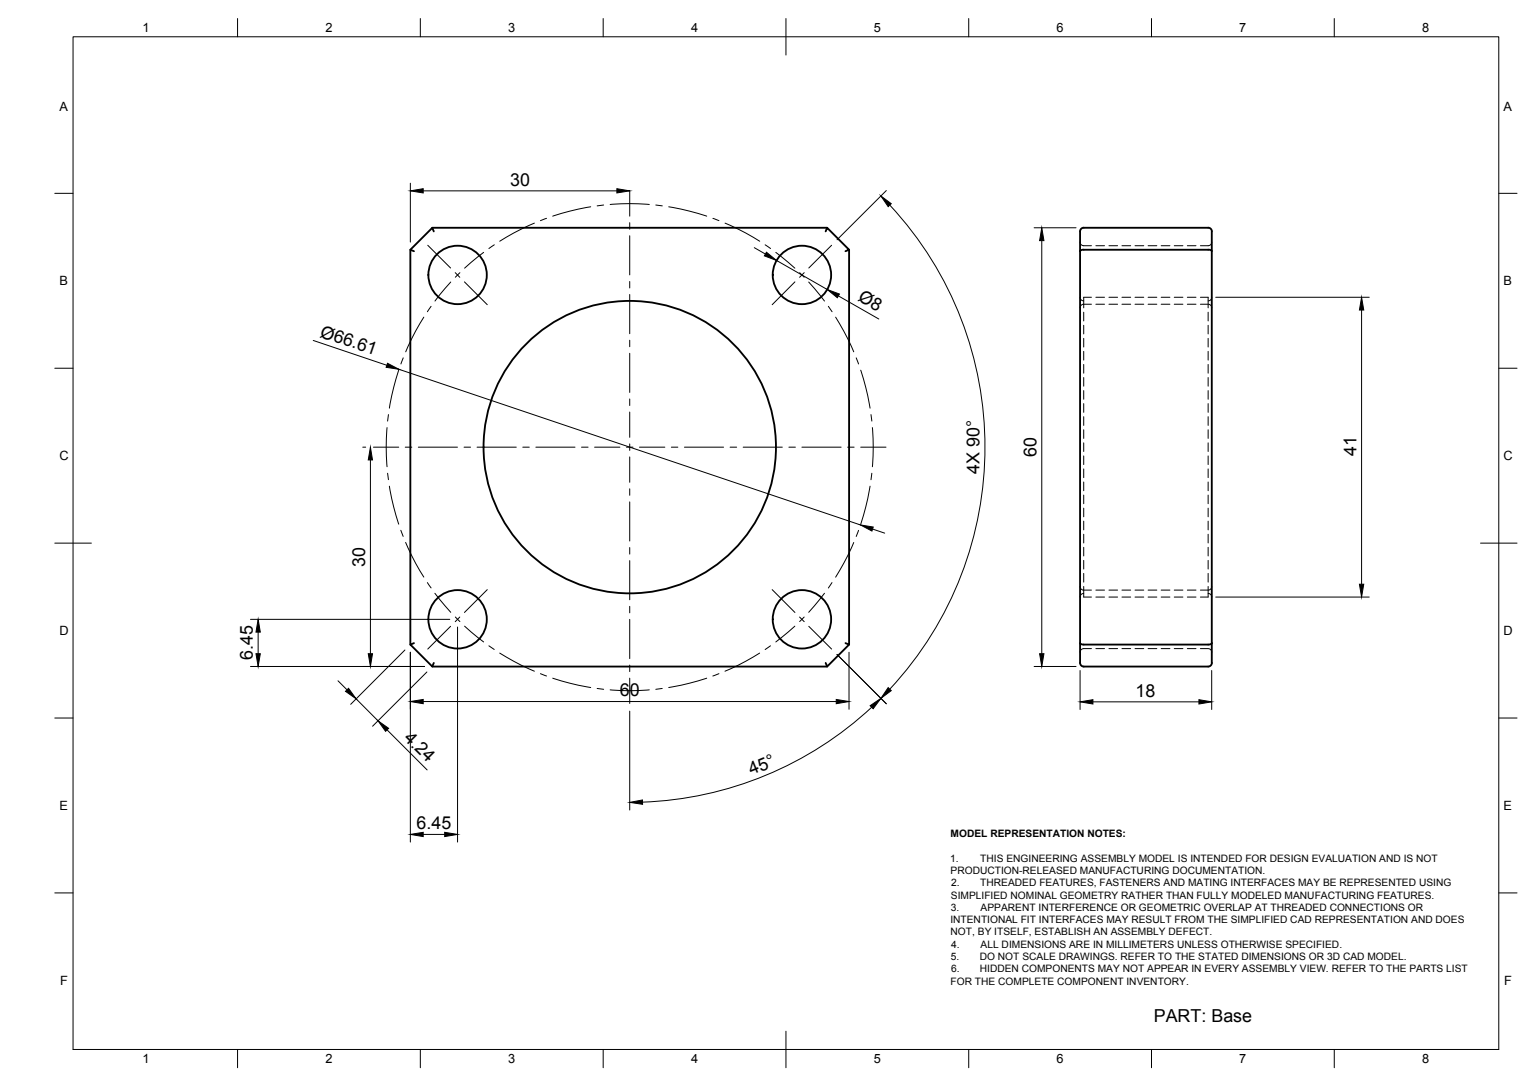
ISO-10303-21;
HEADER;
/* Generated by software containing ST-Developer
 * from STEP Tools, Inc. (www.steptools.com) 
 */

FILE_DESCRIPTION(
/* description */ (''),
/* implementation_level */ '2;1');

FILE_NAME(
/* name */ 'Base.step',
/* time_stamp */ '2026-10-05T14:32:37-07:00',
/* author */ (''),
/* organization */ (''),
/* preprocessor_version */ 'ST-DEVELOPER v20.2',
/* originating_system */ 'Autodesk Translation Framework v15.15.0.0',
/* authorisation */ '');

FILE_SCHEMA (('AUTOMOTIVE_DESIGN { 1 0 10303 214 3 1 1 }'));
ENDSEC;

DATA;
#10=MECHANICAL_DESIGN_GEOMETRIC_PRESENTATION_REPRESENTATION('',(#495),#74103);
#487=SHAPE_REPRESENTATION_RELATIONSHIP('SRR','None',#74129,#491);
#491=ADVANCED_BREP_SHAPE_REPRESENTATION('',(#499),#74100);
#495=STYLED_ITEM('',(#74157),#499);
#499=MANIFOLD_SOLID_BREP('Body1',#4574);
#512=TOROIDAL_SURFACE('',#4736,4.5,0.5);
#513=TOROIDAL_SURFACE('',#4747,4.5,0.5);
#514=TOROIDAL_SURFACE('',#4753,4.5,0.5);
#515=TOROIDAL_SURFACE('',#4759,20.5,0.5);
#516=TOROIDAL_SURFACE('',#4761,4.5,0.5);
#517=TOROIDAL_SURFACE('',#4791,4.5,0.5);
#518=TOROIDAL_SURFACE('',#4799,4.5,0.5);
#519=TOROIDAL_SURFACE('',#4801,20.5,0.5);
#520=TOROIDAL_SURFACE('',#4803,4.5,0.5);
#521=TOROIDAL_SURFACE('',#4821,4.5,0.5);
#542=ELLIPSE('',#4768,0.541196100146197,0.5);
#543=ELLIPSE('',#4769,0.541196100146199,0.5);
#544=ELLIPSE('',#4771,0.541196100146199,0.5);
#545=ELLIPSE('',#4773,0.541196100146197,0.5);
#546=ELLIPSE('',#4775,0.541196100146197,0.5);
#547=ELLIPSE('',#4776,0.541196100146197,0.5);
#548=ELLIPSE('',#4778,0.541196100146199,0.5);
#549=ELLIPSE('',#4781,0.541196100146197,0.5);
#550=ELLIPSE('',#4806,0.541196100146197,0.5);
#551=ELLIPSE('',#4807,0.541196100146198,0.5);
#552=ELLIPSE('',#4809,0.541196100146198,0.5);
#553=ELLIPSE('',#4811,0.541196100146197,0.5);
#554=ELLIPSE('',#4813,0.541196100146197,0.5);
#555=ELLIPSE('',#4814,0.541196100146197,0.5);
#556=ELLIPSE('',#4816,0.541196100146198,0.5);
#557=ELLIPSE('',#4819,0.541196100146197,0.5);
#570=FACE_BOUND('',#856,.T.);
#571=FACE_BOUND('',#858,.T.);
#572=FACE_BOUND('',#861,.T.);
#573=FACE_BOUND('',#862,.T.);
#574=FACE_BOUND('',#863,.T.);
#575=FACE_BOUND('',#864,.T.);
#576=FACE_BOUND('',#865,.T.);
#577=FACE_BOUND('',#892,.T.);
#578=FACE_BOUND('',#893,.T.);
#579=FACE_BOUND('',#894,.T.);
#580=FACE_BOUND('',#895,.T.);
#581=FACE_BOUND('',#896,.T.);
#596=PLANE('',#4730);
#597=PLANE('',#4733);
#598=PLANE('',#4740);
#599=PLANE('',#4783);
#600=PLANE('',#4784);
#601=PLANE('',#4785);
#602=PLANE('',#4786);
#603=PLANE('',#4787);
#604=PLANE('',#4788);
#605=PLANE('',#4789);
#606=PLANE('',#4790);
#607=PLANE('',#4794);
#657=FACE_OUTER_BOUND('',#855,.T.);
#658=FACE_OUTER_BOUND('',#857,.T.);
#659=FACE_OUTER_BOUND('',#859,.T.);
#660=FACE_OUTER_BOUND('',#860,.T.);
#661=FACE_OUTER_BOUND('',#866,.T.);
#662=FACE_OUTER_BOUND('',#867,.T.);
#663=FACE_OUTER_BOUND('',#868,.T.);
#664=FACE_OUTER_BOUND('',#869,.T.);
#665=FACE_OUTER_BOUND('',#870,.T.);
#666=FACE_OUTER_BOUND('',#871,.T.);
#667=FACE_OUTER_BOUND('',#872,.T.);
#668=FACE_OUTER_BOUND('',#873,.T.);
#669=FACE_OUTER_BOUND('',#874,.T.);
#670=FACE_OUTER_BOUND('',#875,.T.);
#671=FACE_OUTER_BOUND('',#876,.T.);
#672=FACE_OUTER_BOUND('',#877,.T.);
#673=FACE_OUTER_BOUND('',#878,.T.);
#674=FACE_OUTER_BOUND('',#879,.T.);
#675=FACE_OUTER_BOUND('',#880,.T.);
#676=FACE_OUTER_BOUND('',#881,.T.);
#677=FACE_OUTER_BOUND('',#882,.T.);
#678=FACE_OUTER_BOUND('',#883,.T.);
#679=FACE_OUTER_BOUND('',#884,.T.);
#680=FACE_OUTER_BOUND('',#885,.T.);
#681=FACE_OUTER_BOUND('',#886,.T.);
#682=FACE_OUTER_BOUND('',#887,.T.);
#683=FACE_OUTER_BOUND('',#888,.T.);
#684=FACE_OUTER_BOUND('',#889,.T.);
#685=FACE_OUTER_BOUND('',#890,.T.);
#686=FACE_OUTER_BOUND('',#891,.T.);
#687=FACE_OUTER_BOUND('',#897,.T.);
#688=FACE_OUTER_BOUND('',#898,.T.);
#689=FACE_OUTER_BOUND('',#899,.T.);
#690=FACE_OUTER_BOUND('',#900,.T.);
#691=FACE_OUTER_BOUND('',#901,.T.);
#692=FACE_OUTER_BOUND('',#902,.T.);
#693=FACE_OUTER_BOUND('',#903,.T.);
#694=FACE_OUTER_BOUND('',#904,.T.);
#695=FACE_OUTER_BOUND('',#905,.T.);
#696=FACE_OUTER_BOUND('',#906,.T.);
#697=FACE_OUTER_BOUND('',#907,.T.);
#698=FACE_OUTER_BOUND('',#908,.T.);
#699=FACE_OUTER_BOUND('',#909,.T.);
#855=EDGE_LOOP('',(#2985));
#856=EDGE_LOOP('',(#2986));
#857=EDGE_LOOP('',(#2987));
#858=EDGE_LOOP('',(#2988));
#859=EDGE_LOOP('',(#2989,#2990,#2991,#2992));
#860=EDGE_LOOP('',(#2993,#2994,#2995,#2996,#2997,#2998,#2999,#3000));
#861=EDGE_LOOP('',(#3001));
#862=EDGE_LOOP('',(#3002));
#863=EDGE_LOOP('',(#3003));
#864=EDGE_LOOP('',(#3004));
#865=EDGE_LOOP('',(#3005));
#866=EDGE_LOOP('',(#3006,#3007,#3008,#3009));
#867=EDGE_LOOP('',(#3010,#3011,#3012,#3013));
#868=EDGE_LOOP('',(#3014,#3015,#3016,#3017,#3018));
#869=EDGE_LOOP('',(#3019,#3020,#3021,#3022));
#870=EDGE_LOOP('',(#3023,#3024,#3025,#3026,#3027));
#871=EDGE_LOOP('',(#3028,#3029,#3030,#3031));
#872=EDGE_LOOP('',(#3032,#3033,#3034,#3035));
#873=EDGE_LOOP('',(#3036,#3037,#3038,#3039,#3040));
#874=EDGE_LOOP('',(#3041,#3042,#3043,#3044));
#875=EDGE_LOOP('',(#3045,#3046,#3047,#3048));
#876=EDGE_LOOP('',(#3049,#3050,#3051,#3052));
#877=EDGE_LOOP('',(#3053,#3054,#3055,#3056));
#878=EDGE_LOOP('',(#3057,#3058,#3059,#3060));
#879=EDGE_LOOP('',(#3061,#3062,#3063,#3064));
#880=EDGE_LOOP('',(#3065,#3066,#3067,#3068));
#881=EDGE_LOOP('',(#3069,#3070,#3071,#3072));
#882=EDGE_LOOP('',(#3073,#3074,#3075,#3076));
#883=EDGE_LOOP('',(#3077,#3078,#3079,#3080));
#884=EDGE_LOOP('',(#3081,#3082,#3083,#3084));
#885=EDGE_LOOP('',(#3085,#3086,#3087,#3088));
#886=EDGE_LOOP('',(#3089,#3090,#3091,#3092));
#887=EDGE_LOOP('',(#3093,#3094,#3095,#3096));
#888=EDGE_LOOP('',(#3097,#3098,#3099,#3100));
#889=EDGE_LOOP('',(#3101,#3102,#3103,#3104));
#890=EDGE_LOOP('',(#3105,#3106,#3107,#3108,#3109));
#891=EDGE_LOOP('',(#3110,#3111,#3112,#3113,#3114,#3115,#3116,#3117));
#892=EDGE_LOOP('',(#3118));
#893=EDGE_LOOP('',(#3119));
#894=EDGE_LOOP('',(#3120));
#895=EDGE_LOOP('',(#3121));
#896=EDGE_LOOP('',(#3122));
#897=EDGE_LOOP('',(#3123,#3124,#3125,#3126,#3127));
#898=EDGE_LOOP('',(#3128,#3129,#3130,#3131));
#899=EDGE_LOOP('',(#3132,#3133,#3134,#3135,#3136));
#900=EDGE_LOOP('',(#3137,#3138,#3139,#3140));
#901=EDGE_LOOP('',(#3141,#3142,#3143,#3144));
#902=EDGE_LOOP('',(#3145,#3146,#3147,#3148));
#903=EDGE_LOOP('',(#3149,#3150,#3151,#3152));
#904=EDGE_LOOP('',(#3153,#3154,#3155,#3156));
#905=EDGE_LOOP('',(#3157,#3158,#3159,#3160));
#906=EDGE_LOOP('',(#3161,#3162,#3163,#3164));
#907=EDGE_LOOP('',(#3165,#3166,#3167,#3168));
#908=EDGE_LOOP('',(#3169,#3170,#3171,#3172));
#909=EDGE_LOOP('',(#3173,#3174,#3175,#3176));
#1057=LINE('',#6015,#1235);
#1058=LINE('',#6017,#1236);
#1059=LINE('',#6019,#1237);
#1060=LINE('',#6021,#1238);
#1061=LINE('',#6023,#1239);
#1062=LINE('',#6025,#1240);
#1063=LINE('',#6027,#1241);
#1064=LINE('',#6028,#1242);
#1065=LINE('',#6039,#1243);
#1066=LINE('',#6047,#1244);
#1067=LINE('',#6057,#1245);
#1068=LINE('',#6069,#1246);
#1069=LINE('',#6077,#1247);
#1070=LINE('',#6082,#1248);
#1071=LINE('',#6086,#1249);
#1072=LINE('',#6091,#1250);
#1073=LINE('',#6095,#1251);
#1074=LINE('',#6098,#1252);
#1075=LINE('',#6101,#1253);
#1076=LINE('',#6104,#1254);
#1077=LINE('',#6107,#1255);
#1078=LINE('',#6109,#1256);
#1079=LINE('',#6110,#1257);
#1080=LINE('',#6113,#1258);
#1081=LINE('',#6114,#1259);
#1082=LINE('',#6117,#1260);
#1083=LINE('',#6118,#1261);
#1084=LINE('',#6121,#1262);
#1085=LINE('',#6122,#1263);
#1086=LINE('',#6125,#1264);
#1087=LINE('',#6127,#1265);
#1088=LINE('',#6128,#1266);
#1089=LINE('',#6130,#1267);
#1090=LINE('',#6133,#1268);
#1091=LINE('',#6134,#1269);
#1092=LINE('',#6136,#1270);
#1093=LINE('',#6144,#1271);
#1094=LINE('',#6146,#1272);
#1095=LINE('',#6148,#1273);
#1096=LINE('',#6150,#1274);
#1097=LINE('',#6152,#1275);
#1098=LINE('',#6154,#1276);
#1099=LINE('',#6156,#1277);
#1100=LINE('',#6157,#1278);
#1101=LINE('',#6191,#1279);
#1235=VECTOR('',#5232,10.);
#1236=VECTOR('',#5233,10.);
#1237=VECTOR('',#5234,10.);
#1238=VECTOR('',#5235,10.);
#1239=VECTOR('',#5236,10.);
#1240=VECTOR('',#5237,10.);
#1241=VECTOR('',#5238,10.);
#1242=VECTOR('',#5239,10.);
#1243=VECTOR('',#5250,4.);
#1244=VECTOR('',#5261,4.);
#1245=VECTOR('',#5274,4.);
#1246=VECTOR('',#5291,4.);
#1247=VECTOR('',#5300,9.99999999999999);
#1248=VECTOR('',#5307,10.);
#1249=VECTOR('',#5312,9.99999999999999);
#1250=VECTOR('',#5317,9.99999999999999);
#1251=VECTOR('',#5322,10.);
#1252=VECTOR('',#5327,10.);
#1253=VECTOR('',#5330,9.99999999999999);
#1254=VECTOR('',#5335,10.);
#1255=VECTOR('',#5338,10.);
#1256=VECTOR('',#5339,10.);
#1257=VECTOR('',#5340,10.);
#1258=VECTOR('',#5343,10.);
#1259=VECTOR('',#5344,9.99999999999999);
#1260=VECTOR('',#5347,10.);
#1261=VECTOR('',#5348,10.);
#1262=VECTOR('',#5351,10.);
#1263=VECTOR('',#5352,9.99999999999999);
#1264=VECTOR('',#5355,10.);
#1265=VECTOR('',#5356,9.99999999999999);
#1266=VECTOR('',#5357,10.);
#1267=VECTOR('',#5360,10.);
#1268=VECTOR('',#5363,10.);
#1269=VECTOR('',#5364,10.);
#1270=VECTOR('',#5367,9.99999999999999);
#1271=VECTOR('',#5376,10.);
#1272=VECTOR('',#5377,10.);
#1273=VECTOR('',#5378,10.);
#1274=VECTOR('',#5379,10.);
#1275=VECTOR('',#5380,10.);
#1276=VECTOR('',#5381,10.);
#1277=VECTOR('',#5382,10.);
#1278=VECTOR('',#5383,10.);
#1279=VECTOR('',#5442,20.5);
#1410=CIRCLE('',#4731,20.5);
#1411=CIRCLE('',#4732,20.);
#1412=CIRCLE('',#4734,20.5);
#1413=CIRCLE('',#4735,20.);
#1414=CIRCLE('',#4737,4.5);
#1415=CIRCLE('',#4738,0.5);
#1416=CIRCLE('',#4739,4.);
#1417=CIRCLE('',#4741,4.5);
#1418=CIRCLE('',#4742,20.5);
#1419=CIRCLE('',#4743,4.5);
#1420=CIRCLE('',#4744,4.5);
#1421=CIRCLE('',#4746,4.);
#1422=CIRCLE('',#4748,0.5);
#1423=CIRCLE('',#4749,4.);
#1424=CIRCLE('',#4751,4.);
#1425=CIRCLE('',#4752,4.);
#1426=CIRCLE('',#4754,0.5);
#1427=CIRCLE('',#4755,4.);
#1428=CIRCLE('',#4757,4.);
#1429=CIRCLE('',#4758,4.);
#1430=CIRCLE('',#4760,0.5);
#1431=CIRCLE('',#4762,0.5);
#1432=CIRCLE('',#4763,4.);
#1433=CIRCLE('',#4765,4.);
#1434=CIRCLE('',#4766,4.);
#1435=CIRCLE('',#4792,4.5);
#1436=CIRCLE('',#4793,0.5);
#1437=CIRCLE('',#4795,4.5);
#1438=CIRCLE('',#4796,4.5);
#1439=CIRCLE('',#4797,4.5);
#1440=CIRCLE('',#4798,20.5);
#1441=CIRCLE('',#4800,0.5);
#1442=CIRCLE('',#4802,0.5);
#1443=CIRCLE('',#4804,0.5);
#1444=CIRCLE('',#4822,0.5);
#1527=VERTEX_POINT('',#5997);
#1528=VERTEX_POINT('',#5999);
#1529=VERTEX_POINT('',#6002);
#1530=VERTEX_POINT('',#6004);
#1531=VERTEX_POINT('',#6007);
#1532=VERTEX_POINT('',#6009);
#1533=VERTEX_POINT('',#6013);
#1534=VERTEX_POINT('',#6014);
#1535=VERTEX_POINT('',#6016);
#1536=VERTEX_POINT('',#6018);
#1537=VERTEX_POINT('',#6020);
#1538=VERTEX_POINT('',#6022);
#1539=VERTEX_POINT('',#6024);
#1540=VERTEX_POINT('',#6026);
#1541=VERTEX_POINT('',#6029);
#1542=VERTEX_POINT('',#6031);
#1543=VERTEX_POINT('',#6033);
#1544=VERTEX_POINT('',#6035);
#1545=VERTEX_POINT('',#6038);
#1546=VERTEX_POINT('',#6042);
#1547=VERTEX_POINT('',#6046);
#1548=VERTEX_POINT('',#6048);
#1549=VERTEX_POINT('',#6052);
#1550=VERTEX_POINT('',#6056);
#1551=VERTEX_POINT('',#6058);
#1552=VERTEX_POINT('',#6064);
#1553=VERTEX_POINT('',#6068);
#1554=VERTEX_POINT('',#6070);
#1555=VERTEX_POINT('',#6074);
#1556=VERTEX_POINT('',#6076);
#1557=VERTEX_POINT('',#6080);
#1558=VERTEX_POINT('',#6084);
#1559=VERTEX_POINT('',#6088);
#1560=VERTEX_POINT('',#6090);
#1561=VERTEX_POINT('',#6094);
#1562=VERTEX_POINT('',#6100);
#1563=VERTEX_POINT('',#6106);
#1564=VERTEX_POINT('',#6108);
#1565=VERTEX_POINT('',#6112);
#1566=VERTEX_POINT('',#6116);
#1567=VERTEX_POINT('',#6120);
#1568=VERTEX_POINT('',#6124);
#1569=VERTEX_POINT('',#6126);
#1570=VERTEX_POINT('',#6132);
#1571=VERTEX_POINT('',#6138);
#1572=VERTEX_POINT('',#6142);
#1573=VERTEX_POINT('',#6143);
#1574=VERTEX_POINT('',#6145);
#1575=VERTEX_POINT('',#6147);
#1576=VERTEX_POINT('',#6149);
#1577=VERTEX_POINT('',#6151);
#1578=VERTEX_POINT('',#6153);
#1579=VERTEX_POINT('',#6155);
#1580=VERTEX_POINT('',#6158);
#1581=VERTEX_POINT('',#6160);
#1582=VERTEX_POINT('',#6162);
#1583=VERTEX_POINT('',#6164);
#2136=EDGE_CURVE('',#1527,#1527,#1410,.T.);
#2137=EDGE_CURVE('',#1528,#1528,#1411,.T.);
#2138=EDGE_CURVE('',#1529,#1529,#1412,.T.);
#2139=EDGE_CURVE('',#1530,#1530,#1413,.T.);
#2140=EDGE_CURVE('',#1531,#1531,#1414,.T.);
#2141=EDGE_CURVE('',#1531,#1532,#1415,.T.);
#2142=EDGE_CURVE('',#1532,#1532,#1416,.T.);
#2143=EDGE_CURVE('',#1533,#1534,#1057,.T.);
#2144=EDGE_CURVE('',#1535,#1533,#1058,.T.);
#2145=EDGE_CURVE('',#1536,#1535,#1059,.T.);
#2146=EDGE_CURVE('',#1537,#1536,#1060,.T.);
#2147=EDGE_CURVE('',#1538,#1537,#1061,.T.);
#2148=EDGE_CURVE('',#1539,#1538,#1062,.T.);
#2149=EDGE_CURVE('',#1540,#1539,#1063,.T.);
#2150=EDGE_CURVE('',#1534,#1540,#1064,.T.);
#2151=EDGE_CURVE('',#1541,#1541,#1417,.T.);
#2152=EDGE_CURVE('',#1542,#1542,#1418,.T.);
#2153=EDGE_CURVE('',#1543,#1543,#1419,.T.);
#2154=EDGE_CURVE('',#1544,#1544,#1420,.T.);
#2155=EDGE_CURVE('',#1532,#1545,#1065,.T.);
#2156=EDGE_CURVE('',#1545,#1545,#1421,.T.);
#2157=EDGE_CURVE('',#1541,#1546,#1422,.T.);
#2158=EDGE_CURVE('',#1546,#1546,#1423,.T.);
#2159=EDGE_CURVE('',#1546,#1547,#1066,.T.);
#2160=EDGE_CURVE('',#1548,#1547,#1424,.T.);
#2161=EDGE_CURVE('',#1547,#1548,#1425,.T.);
#2162=EDGE_CURVE('',#1544,#1549,#1426,.T.);
#2163=EDGE_CURVE('',#1549,#1549,#1427,.T.);
#2164=EDGE_CURVE('',#1549,#1550,#1067,.T.);
#2165=EDGE_CURVE('',#1551,#1550,#1428,.T.);
#2166=EDGE_CURVE('',#1550,#1551,#1429,.T.);
#2167=EDGE_CURVE('',#1542,#1528,#1430,.T.);
#2168=EDGE_CURVE('',#1543,#1552,#1431,.T.);
#2169=EDGE_CURVE('',#1552,#1552,#1432,.T.);
#2170=EDGE_CURVE('',#1552,#1553,#1068,.T.);
#2171=EDGE_CURVE('',#1554,#1553,#1433,.T.);
#2172=EDGE_CURVE('',#1553,#1554,#1434,.T.);
#2173=EDGE_CURVE('',#1537,#1555,#542,.T.);
#2174=EDGE_CURVE('',#1555,#1556,#1069,.T.);
#2175=EDGE_CURVE('',#1538,#1556,#543,.T.);
#2176=EDGE_CURVE('',#1536,#1557,#544,.T.);
#2177=EDGE_CURVE('',#1557,#1555,#1070,.T.);
#2178=EDGE_CURVE('',#1535,#1558,#545,.T.);
#2179=EDGE_CURVE('',#1558,#1557,#1071,.T.);
#2180=EDGE_CURVE('',#1534,#1559,#546,.T.);
#2181=EDGE_CURVE('',#1559,#1560,#1072,.T.);
#2182=EDGE_CURVE('',#1560,#1533,#547,.T.);
#2183=EDGE_CURVE('',#1561,#1559,#1073,.T.);
#2184=EDGE_CURVE('',#1540,#1561,#548,.T.);
#2185=EDGE_CURVE('',#1560,#1558,#1074,.T.);
#2186=EDGE_CURVE('',#1562,#1561,#1075,.T.);
#2187=EDGE_CURVE('',#1539,#1562,#549,.T.);
#2188=EDGE_CURVE('',#1556,#1562,#1076,.T.);
#2189=EDGE_CURVE('',#1557,#1563,#1077,.T.);
#2190=EDGE_CURVE('',#1564,#1563,#1078,.T.);
#2191=EDGE_CURVE('',#1555,#1564,#1079,.T.);
#2192=EDGE_CURVE('',#1558,#1565,#1080,.T.);
#2193=EDGE_CURVE('',#1563,#1565,#1081,.T.);
#2194=EDGE_CURVE('',#1560,#1566,#1082,.T.);
#2195=EDGE_CURVE('',#1565,#1566,#1083,.T.);
#2196=EDGE_CURVE('',#1559,#1567,#1084,.T.);
#2197=EDGE_CURVE('',#1566,#1567,#1085,.T.);
#2198=EDGE_CURVE('',#1562,#1568,#1086,.T.);
#2199=EDGE_CURVE('',#1569,#1568,#1087,.T.);
#2200=EDGE_CURVE('',#1561,#1569,#1088,.T.);
#2201=EDGE_CURVE('',#1567,#1569,#1089,.T.);
#2202=EDGE_CURVE('',#1556,#1570,#1090,.T.);
#2203=EDGE_CURVE('',#1568,#1570,#1091,.T.);
#2204=EDGE_CURVE('',#1570,#1564,#1092,.T.);
#2205=EDGE_CURVE('',#1571,#1571,#1435,.T.);
#2206=EDGE_CURVE('',#1571,#1548,#1436,.T.);
#2207=EDGE_CURVE('',#1572,#1573,#1093,.T.);
#2208=EDGE_CURVE('',#1574,#1572,#1094,.T.);
#2209=EDGE_CURVE('',#1575,#1574,#1095,.T.);
#2210=EDGE_CURVE('',#1576,#1575,#1096,.T.);
#2211=EDGE_CURVE('',#1577,#1576,#1097,.T.);
#2212=EDGE_CURVE('',#1578,#1577,#1098,.T.);
#2213=EDGE_CURVE('',#1579,#1578,#1099,.T.);
#2214=EDGE_CURVE('',#1573,#1579,#1100,.T.);
#2215=EDGE_CURVE('',#1580,#1580,#1437,.T.);
#2216=EDGE_CURVE('',#1581,#1581,#1438,.T.);
#2217=EDGE_CURVE('',#1582,#1582,#1439,.T.);
#2218=EDGE_CURVE('',#1583,#1583,#1440,.T.);
#2219=EDGE_CURVE('',#1580,#1551,#1441,.T.);
#2220=EDGE_CURVE('',#1583,#1530,#1442,.T.);
#2221=EDGE_CURVE('',#1581,#1554,#1443,.T.);
#2222=EDGE_CURVE('',#1576,#1563,#550,.T.);
#2223=EDGE_CURVE('',#1577,#1565,#551,.T.);
#2224=EDGE_CURVE('',#1575,#1564,#552,.T.);
#2225=EDGE_CURVE('',#1574,#1570,#553,.T.);
#2226=EDGE_CURVE('',#1573,#1569,#554,.T.);
#2227=EDGE_CURVE('',#1568,#1572,#555,.T.);
#2228=EDGE_CURVE('',#1579,#1567,#556,.T.);
#2229=EDGE_CURVE('',#1578,#1566,#557,.T.);
#2230=EDGE_CURVE('',#1545,#1582,#1444,.T.);
#2231=EDGE_CURVE('',#1527,#1529,#1101,.T.);
#2985=ORIENTED_EDGE('',*,*,#2136,.T.);
#2986=ORIENTED_EDGE('',*,*,#2137,.F.);
#2987=ORIENTED_EDGE('',*,*,#2138,.F.);
#2988=ORIENTED_EDGE('',*,*,#2139,.F.);
#2989=ORIENTED_EDGE('',*,*,#2140,.T.);
#2990=ORIENTED_EDGE('',*,*,#2141,.T.);
#2991=ORIENTED_EDGE('',*,*,#2142,.T.);
#2992=ORIENTED_EDGE('',*,*,#2141,.F.);
#2993=ORIENTED_EDGE('',*,*,#2143,.F.);
#2994=ORIENTED_EDGE('',*,*,#2144,.F.);
#2995=ORIENTED_EDGE('',*,*,#2145,.F.);
#2996=ORIENTED_EDGE('',*,*,#2146,.F.);
#2997=ORIENTED_EDGE('',*,*,#2147,.F.);
#2998=ORIENTED_EDGE('',*,*,#2148,.F.);
#2999=ORIENTED_EDGE('',*,*,#2149,.F.);
#3000=ORIENTED_EDGE('',*,*,#2150,.F.);
#3001=ORIENTED_EDGE('',*,*,#2151,.F.);
#3002=ORIENTED_EDGE('',*,*,#2152,.F.);
#3003=ORIENTED_EDGE('',*,*,#2153,.F.);
#3004=ORIENTED_EDGE('',*,*,#2154,.F.);
#3005=ORIENTED_EDGE('',*,*,#2140,.F.);
#3006=ORIENTED_EDGE('',*,*,#2142,.F.);
#3007=ORIENTED_EDGE('',*,*,#2155,.T.);
#3008=ORIENTED_EDGE('',*,*,#2156,.F.);
#3009=ORIENTED_EDGE('',*,*,#2155,.F.);
#3010=ORIENTED_EDGE('',*,*,#2151,.T.);
#3011=ORIENTED_EDGE('',*,*,#2157,.T.);
#3012=ORIENTED_EDGE('',*,*,#2158,.T.);
#3013=ORIENTED_EDGE('',*,*,#2157,.F.);
#3014=ORIENTED_EDGE('',*,*,#2158,.F.);
#3015=ORIENTED_EDGE('',*,*,#2159,.T.);
#3016=ORIENTED_EDGE('',*,*,#2160,.F.);
#3017=ORIENTED_EDGE('',*,*,#2161,.F.);
#3018=ORIENTED_EDGE('',*,*,#2159,.F.);
#3019=ORIENTED_EDGE('',*,*,#2154,.T.);
#3020=ORIENTED_EDGE('',*,*,#2162,.T.);
#3021=ORIENTED_EDGE('',*,*,#2163,.T.);
#3022=ORIENTED_EDGE('',*,*,#2162,.F.);
#3023=ORIENTED_EDGE('',*,*,#2163,.F.);
#3024=ORIENTED_EDGE('',*,*,#2164,.T.);
#3025=ORIENTED_EDGE('',*,*,#2165,.F.);
#3026=ORIENTED_EDGE('',*,*,#2166,.F.);
#3027=ORIENTED_EDGE('',*,*,#2164,.F.);
#3028=ORIENTED_EDGE('',*,*,#2152,.T.);
#3029=ORIENTED_EDGE('',*,*,#2167,.T.);
#3030=ORIENTED_EDGE('',*,*,#2137,.T.);
#3031=ORIENTED_EDGE('',*,*,#2167,.F.);
#3032=ORIENTED_EDGE('',*,*,#2153,.T.);
#3033=ORIENTED_EDGE('',*,*,#2168,.T.);
#3034=ORIENTED_EDGE('',*,*,#2169,.T.);
#3035=ORIENTED_EDGE('',*,*,#2168,.F.);
#3036=ORIENTED_EDGE('',*,*,#2169,.F.);
#3037=ORIENTED_EDGE('',*,*,#2170,.T.);
#3038=ORIENTED_EDGE('',*,*,#2171,.F.);
#3039=ORIENTED_EDGE('',*,*,#2172,.F.);
#3040=ORIENTED_EDGE('',*,*,#2170,.F.);
#3041=ORIENTED_EDGE('',*,*,#2147,.T.);
#3042=ORIENTED_EDGE('',*,*,#2173,.T.);
#3043=ORIENTED_EDGE('',*,*,#2174,.T.);
#3044=ORIENTED_EDGE('',*,*,#2175,.F.);
#3045=ORIENTED_EDGE('',*,*,#2146,.T.);
#3046=ORIENTED_EDGE('',*,*,#2176,.T.);
#3047=ORIENTED_EDGE('',*,*,#2177,.T.);
#3048=ORIENTED_EDGE('',*,*,#2173,.F.);
#3049=ORIENTED_EDGE('',*,*,#2145,.T.);
#3050=ORIENTED_EDGE('',*,*,#2178,.T.);
#3051=ORIENTED_EDGE('',*,*,#2179,.T.);
#3052=ORIENTED_EDGE('',*,*,#2176,.F.);
#3053=ORIENTED_EDGE('',*,*,#2143,.T.);
#3054=ORIENTED_EDGE('',*,*,#2180,.T.);
#3055=ORIENTED_EDGE('',*,*,#2181,.T.);
#3056=ORIENTED_EDGE('',*,*,#2182,.T.);
#3057=ORIENTED_EDGE('',*,*,#2183,.T.);
#3058=ORIENTED_EDGE('',*,*,#2180,.F.);
#3059=ORIENTED_EDGE('',*,*,#2150,.T.);
#3060=ORIENTED_EDGE('',*,*,#2184,.T.);
#3061=ORIENTED_EDGE('',*,*,#2144,.T.);
#3062=ORIENTED_EDGE('',*,*,#2182,.F.);
#3063=ORIENTED_EDGE('',*,*,#2185,.T.);
#3064=ORIENTED_EDGE('',*,*,#2178,.F.);
#3065=ORIENTED_EDGE('',*,*,#2186,.T.);
#3066=ORIENTED_EDGE('',*,*,#2184,.F.);
#3067=ORIENTED_EDGE('',*,*,#2149,.T.);
#3068=ORIENTED_EDGE('',*,*,#2187,.T.);
#3069=ORIENTED_EDGE('',*,*,#2188,.T.);
#3070=ORIENTED_EDGE('',*,*,#2187,.F.);
#3071=ORIENTED_EDGE('',*,*,#2148,.T.);
#3072=ORIENTED_EDGE('',*,*,#2175,.T.);
#3073=ORIENTED_EDGE('',*,*,#2177,.F.);
#3074=ORIENTED_EDGE('',*,*,#2189,.T.);
#3075=ORIENTED_EDGE('',*,*,#2190,.F.);
#3076=ORIENTED_EDGE('',*,*,#2191,.F.);
#3077=ORIENTED_EDGE('',*,*,#2179,.F.);
#3078=ORIENTED_EDGE('',*,*,#2192,.T.);
#3079=ORIENTED_EDGE('',*,*,#2193,.F.);
#3080=ORIENTED_EDGE('',*,*,#2189,.F.);
#3081=ORIENTED_EDGE('',*,*,#2185,.F.);
#3082=ORIENTED_EDGE('',*,*,#2194,.T.);
#3083=ORIENTED_EDGE('',*,*,#2195,.F.);
#3084=ORIENTED_EDGE('',*,*,#2192,.F.);
#3085=ORIENTED_EDGE('',*,*,#2181,.F.);
#3086=ORIENTED_EDGE('',*,*,#2196,.T.);
#3087=ORIENTED_EDGE('',*,*,#2197,.F.);
#3088=ORIENTED_EDGE('',*,*,#2194,.F.);
#3089=ORIENTED_EDGE('',*,*,#2186,.F.);
#3090=ORIENTED_EDGE('',*,*,#2198,.T.);
#3091=ORIENTED_EDGE('',*,*,#2199,.F.);
#3092=ORIENTED_EDGE('',*,*,#2200,.F.);
#3093=ORIENTED_EDGE('',*,*,#2183,.F.);
#3094=ORIENTED_EDGE('',*,*,#2200,.T.);
#3095=ORIENTED_EDGE('',*,*,#2201,.F.);
#3096=ORIENTED_EDGE('',*,*,#2196,.F.);
#3097=ORIENTED_EDGE('',*,*,#2188,.F.);
#3098=ORIENTED_EDGE('',*,*,#2202,.T.);
#3099=ORIENTED_EDGE('',*,*,#2203,.F.);
#3100=ORIENTED_EDGE('',*,*,#2198,.F.);
#3101=ORIENTED_EDGE('',*,*,#2174,.F.);
#3102=ORIENTED_EDGE('',*,*,#2191,.T.);
#3103=ORIENTED_EDGE('',*,*,#2204,.F.);
#3104=ORIENTED_EDGE('',*,*,#2202,.F.);
#3105=ORIENTED_EDGE('',*,*,#2205,.T.);
#3106=ORIENTED_EDGE('',*,*,#2206,.T.);
#3107=ORIENTED_EDGE('',*,*,#2160,.T.);
#3108=ORIENTED_EDGE('',*,*,#2161,.T.);
#3109=ORIENTED_EDGE('',*,*,#2206,.F.);
#3110=ORIENTED_EDGE('',*,*,#2207,.F.);
#3111=ORIENTED_EDGE('',*,*,#2208,.F.);
#3112=ORIENTED_EDGE('',*,*,#2209,.F.);
#3113=ORIENTED_EDGE('',*,*,#2210,.F.);
#3114=ORIENTED_EDGE('',*,*,#2211,.F.);
#3115=ORIENTED_EDGE('',*,*,#2212,.F.);
#3116=ORIENTED_EDGE('',*,*,#2213,.F.);
#3117=ORIENTED_EDGE('',*,*,#2214,.F.);
#3118=ORIENTED_EDGE('',*,*,#2215,.F.);
#3119=ORIENTED_EDGE('',*,*,#2216,.F.);
#3120=ORIENTED_EDGE('',*,*,#2217,.F.);
#3121=ORIENTED_EDGE('',*,*,#2218,.F.);
#3122=ORIENTED_EDGE('',*,*,#2205,.F.);
#3123=ORIENTED_EDGE('',*,*,#2215,.T.);
#3124=ORIENTED_EDGE('',*,*,#2219,.T.);
#3125=ORIENTED_EDGE('',*,*,#2165,.T.);
#3126=ORIENTED_EDGE('',*,*,#2166,.T.);
#3127=ORIENTED_EDGE('',*,*,#2219,.F.);
#3128=ORIENTED_EDGE('',*,*,#2218,.T.);
#3129=ORIENTED_EDGE('',*,*,#2220,.T.);
#3130=ORIENTED_EDGE('',*,*,#2139,.T.);
#3131=ORIENTED_EDGE('',*,*,#2220,.F.);
#3132=ORIENTED_EDGE('',*,*,#2216,.T.);
#3133=ORIENTED_EDGE('',*,*,#2221,.T.);
#3134=ORIENTED_EDGE('',*,*,#2171,.T.);
#3135=ORIENTED_EDGE('',*,*,#2172,.T.);
#3136=ORIENTED_EDGE('',*,*,#2221,.F.);
#3137=ORIENTED_EDGE('',*,*,#2211,.T.);
#3138=ORIENTED_EDGE('',*,*,#2222,.T.);
#3139=ORIENTED_EDGE('',*,*,#2193,.T.);
#3140=ORIENTED_EDGE('',*,*,#2223,.F.);
#3141=ORIENTED_EDGE('',*,*,#2210,.T.);
#3142=ORIENTED_EDGE('',*,*,#2224,.T.);
#3143=ORIENTED_EDGE('',*,*,#2190,.T.);
#3144=ORIENTED_EDGE('',*,*,#2222,.F.);
#3145=ORIENTED_EDGE('',*,*,#2209,.T.);
#3146=ORIENTED_EDGE('',*,*,#2225,.T.);
#3147=ORIENTED_EDGE('',*,*,#2204,.T.);
#3148=ORIENTED_EDGE('',*,*,#2224,.F.);
#3149=ORIENTED_EDGE('',*,*,#2207,.T.);
#3150=ORIENTED_EDGE('',*,*,#2226,.T.);
#3151=ORIENTED_EDGE('',*,*,#2199,.T.);
#3152=ORIENTED_EDGE('',*,*,#2227,.T.);
#3153=ORIENTED_EDGE('',*,*,#2201,.T.);
#3154=ORIENTED_EDGE('',*,*,#2226,.F.);
#3155=ORIENTED_EDGE('',*,*,#2214,.T.);
#3156=ORIENTED_EDGE('',*,*,#2228,.T.);
#3157=ORIENTED_EDGE('',*,*,#2208,.T.);
#3158=ORIENTED_EDGE('',*,*,#2227,.F.);
#3159=ORIENTED_EDGE('',*,*,#2203,.T.);
#3160=ORIENTED_EDGE('',*,*,#2225,.F.);
#3161=ORIENTED_EDGE('',*,*,#2197,.T.);
#3162=ORIENTED_EDGE('',*,*,#2228,.F.);
#3163=ORIENTED_EDGE('',*,*,#2213,.T.);
#3164=ORIENTED_EDGE('',*,*,#2229,.T.);
#3165=ORIENTED_EDGE('',*,*,#2195,.T.);
#3166=ORIENTED_EDGE('',*,*,#2229,.F.);
#3167=ORIENTED_EDGE('',*,*,#2212,.T.);
#3168=ORIENTED_EDGE('',*,*,#2223,.T.);
#3169=ORIENTED_EDGE('',*,*,#2156,.T.);
#3170=ORIENTED_EDGE('',*,*,#2230,.T.);
#3171=ORIENTED_EDGE('',*,*,#2217,.T.);
#3172=ORIENTED_EDGE('',*,*,#2230,.F.);
#3173=ORIENTED_EDGE('',*,*,#2136,.F.);
#3174=ORIENTED_EDGE('',*,*,#2231,.T.);
#3175=ORIENTED_EDGE('',*,*,#2138,.T.);
#3176=ORIENTED_EDGE('',*,*,#2231,.F.);
#4278=CYLINDRICAL_SURFACE('',#4745,4.);
#4279=CYLINDRICAL_SURFACE('',#4750,4.);
#4280=CYLINDRICAL_SURFACE('',#4756,4.);
#4281=CYLINDRICAL_SURFACE('',#4764,4.);
#4282=CYLINDRICAL_SURFACE('',#4767,0.5);
#4283=CYLINDRICAL_SURFACE('',#4770,0.5);
#4284=CYLINDRICAL_SURFACE('',#4772,0.5);
#4285=CYLINDRICAL_SURFACE('',#4774,0.5);
#4286=CYLINDRICAL_SURFACE('',#4777,0.5);
#4287=CYLINDRICAL_SURFACE('',#4779,0.5);
#4288=CYLINDRICAL_SURFACE('',#4780,0.5);
#4289=CYLINDRICAL_SURFACE('',#4782,0.5);
#4290=CYLINDRICAL_SURFACE('',#4805,0.5);
#4291=CYLINDRICAL_SURFACE('',#4808,0.5);
#4292=CYLINDRICAL_SURFACE('',#4810,0.5);
#4293=CYLINDRICAL_SURFACE('',#4812,0.5);
#4294=CYLINDRICAL_SURFACE('',#4815,0.5);
#4295=CYLINDRICAL_SURFACE('',#4817,0.5);
#4296=CYLINDRICAL_SURFACE('',#4818,0.5);
#4297=CYLINDRICAL_SURFACE('',#4820,0.5);
#4298=CYLINDRICAL_SURFACE('',#4823,20.5);
#4432=ADVANCED_FACE('',(#657,#570),#596,.F.);
#4433=ADVANCED_FACE('',(#658,#571),#597,.F.);
#4434=ADVANCED_FACE('',(#659),#512,.T.);
#4435=ADVANCED_FACE('',(#660,#572,#573,#574,#575,#576),#598,.F.);
#4436=ADVANCED_FACE('',(#661),#4278,.F.);
#4437=ADVANCED_FACE('',(#662),#513,.T.);
#4438=ADVANCED_FACE('',(#663),#4279,.F.);
#4439=ADVANCED_FACE('',(#664),#514,.T.);
#4440=ADVANCED_FACE('',(#665),#4280,.F.);
#4441=ADVANCED_FACE('',(#666),#515,.T.);
#4442=ADVANCED_FACE('',(#667),#516,.T.);
#4443=ADVANCED_FACE('',(#668),#4281,.F.);
#4444=ADVANCED_FACE('',(#669),#4282,.T.);
#4445=ADVANCED_FACE('',(#670),#4283,.T.);
#4446=ADVANCED_FACE('',(#671),#4284,.T.);
#4447=ADVANCED_FACE('',(#672),#4285,.T.);
#4448=ADVANCED_FACE('',(#673),#4286,.T.);
#4449=ADVANCED_FACE('',(#674),#4287,.T.);
#4450=ADVANCED_FACE('',(#675),#4288,.T.);
#4451=ADVANCED_FACE('',(#676),#4289,.T.);
#4452=ADVANCED_FACE('',(#677),#599,.T.);
#4453=ADVANCED_FACE('',(#678),#600,.T.);
#4454=ADVANCED_FACE('',(#679),#601,.T.);
#4455=ADVANCED_FACE('',(#680),#602,.T.);
#4456=ADVANCED_FACE('',(#681),#603,.T.);
#4457=ADVANCED_FACE('',(#682),#604,.T.);
#4458=ADVANCED_FACE('',(#683),#605,.T.);
#4459=ADVANCED_FACE('',(#684),#606,.T.);
#4460=ADVANCED_FACE('',(#685),#517,.T.);
#4461=ADVANCED_FACE('',(#686,#577,#578,#579,#580,#581),#607,.T.);
#4462=ADVANCED_FACE('',(#687),#518,.T.);
#4463=ADVANCED_FACE('',(#688),#519,.T.);
#4464=ADVANCED_FACE('',(#689),#520,.T.);
#4465=ADVANCED_FACE('',(#690),#4290,.T.);
#4466=ADVANCED_FACE('',(#691),#4291,.T.);
#4467=ADVANCED_FACE('',(#692),#4292,.T.);
#4468=ADVANCED_FACE('',(#693),#4293,.T.);
#4469=ADVANCED_FACE('',(#694),#4294,.T.);
#4470=ADVANCED_FACE('',(#695),#4295,.T.);
#4471=ADVANCED_FACE('',(#696),#4296,.T.);
#4472=ADVANCED_FACE('',(#697),#4297,.T.);
#4473=ADVANCED_FACE('',(#698),#521,.T.);
#4474=ADVANCED_FACE('',(#699),#4298,.F.);
#4574=CLOSED_SHELL('',(#4432,#4433,#4434,#4435,#4436,#4437,#4438,#4439,
#4440,#4441,#4442,#4443,#4444,#4445,#4446,#4447,#4448,#4449,#4450,#4451,
#4452,#4453,#4454,#4455,#4456,#4457,#4458,#4459,#4460,#4461,#4462,#4463,
#4464,#4465,#4466,#4467,#4468,#4469,#4470,#4471,#4472,#4473,#4474));
#4729=AXIS2_PLACEMENT_3D('',#5995,#5208,#5209);
#4730=AXIS2_PLACEMENT_3D('',#5996,#5210,#5211);
#4731=AXIS2_PLACEMENT_3D('',#5998,#5212,#5213);
#4732=AXIS2_PLACEMENT_3D('',#6000,#5214,#5215);
#4733=AXIS2_PLACEMENT_3D('',#6001,#5216,#5217);
#4734=AXIS2_PLACEMENT_3D('',#6003,#5218,#5219);
#4735=AXIS2_PLACEMENT_3D('',#6005,#5220,#5221);
#4736=AXIS2_PLACEMENT_3D('',#6006,#5222,#5223);
#4737=AXIS2_PLACEMENT_3D('',#6008,#5224,#5225);
#4738=AXIS2_PLACEMENT_3D('',#6010,#5226,#5227);
#4739=AXIS2_PLACEMENT_3D('',#6011,#5228,#5229);
#4740=AXIS2_PLACEMENT_3D('',#6012,#5230,#5231);
#4741=AXIS2_PLACEMENT_3D('',#6030,#5240,#5241);
#4742=AXIS2_PLACEMENT_3D('',#6032,#5242,#5243);
#4743=AXIS2_PLACEMENT_3D('',#6034,#5244,#5245);
#4744=AXIS2_PLACEMENT_3D('',#6036,#5246,#5247);
#4745=AXIS2_PLACEMENT_3D('',#6037,#5248,#5249);
#4746=AXIS2_PLACEMENT_3D('',#6040,#5251,#5252);
#4747=AXIS2_PLACEMENT_3D('',#6041,#5253,#5254);
#4748=AXIS2_PLACEMENT_3D('',#6043,#5255,#5256);
#4749=AXIS2_PLACEMENT_3D('',#6044,#5257,#5258);
#4750=AXIS2_PLACEMENT_3D('',#6045,#5259,#5260);
#4751=AXIS2_PLACEMENT_3D('',#6049,#5262,#5263);
#4752=AXIS2_PLACEMENT_3D('',#6050,#5264,#5265);
#4753=AXIS2_PLACEMENT_3D('',#6051,#5266,#5267);
#4754=AXIS2_PLACEMENT_3D('',#6053,#5268,#5269);
#4755=AXIS2_PLACEMENT_3D('',#6054,#5270,#5271);
#4756=AXIS2_PLACEMENT_3D('',#6055,#5272,#5273);
#4757=AXIS2_PLACEMENT_3D('',#6059,#5275,#5276);
#4758=AXIS2_PLACEMENT_3D('',#6060,#5277,#5278);
#4759=AXIS2_PLACEMENT_3D('',#6061,#5279,#5280);
#4760=AXIS2_PLACEMENT_3D('',#6062,#5281,#5282);
#4761=AXIS2_PLACEMENT_3D('',#6063,#5283,#5284);
#4762=AXIS2_PLACEMENT_3D('',#6065,#5285,#5286);
#4763=AXIS2_PLACEMENT_3D('',#6066,#5287,#5288);
#4764=AXIS2_PLACEMENT_3D('',#6067,#5289,#5290);
#4765=AXIS2_PLACEMENT_3D('',#6071,#5292,#5293);
#4766=AXIS2_PLACEMENT_3D('',#6072,#5294,#5295);
#4767=AXIS2_PLACEMENT_3D('',#6073,#5296,#5297);
#4768=AXIS2_PLACEMENT_3D('',#6075,#5298,#5299);
#4769=AXIS2_PLACEMENT_3D('',#6078,#5301,#5302);
#4770=AXIS2_PLACEMENT_3D('',#6079,#5303,#5304);
#4771=AXIS2_PLACEMENT_3D('',#6081,#5305,#5306);
#4772=AXIS2_PLACEMENT_3D('',#6083,#5308,#5309);
#4773=AXIS2_PLACEMENT_3D('',#6085,#5310,#5311);
#4774=AXIS2_PLACEMENT_3D('',#6087,#5313,#5314);
#4775=AXIS2_PLACEMENT_3D('',#6089,#5315,#5316);
#4776=AXIS2_PLACEMENT_3D('',#6092,#5318,#5319);
#4777=AXIS2_PLACEMENT_3D('',#6093,#5320,#5321);
#4778=AXIS2_PLACEMENT_3D('',#6096,#5323,#5324);
#4779=AXIS2_PLACEMENT_3D('',#6097,#5325,#5326);
#4780=AXIS2_PLACEMENT_3D('',#6099,#5328,#5329);
#4781=AXIS2_PLACEMENT_3D('',#6102,#5331,#5332);
#4782=AXIS2_PLACEMENT_3D('',#6103,#5333,#5334);
#4783=AXIS2_PLACEMENT_3D('',#6105,#5336,#5337);
#4784=AXIS2_PLACEMENT_3D('',#6111,#5341,#5342);
#4785=AXIS2_PLACEMENT_3D('',#6115,#5345,#5346);
#4786=AXIS2_PLACEMENT_3D('',#6119,#5349,#5350);
#4787=AXIS2_PLACEMENT_3D('',#6123,#5353,#5354);
#4788=AXIS2_PLACEMENT_3D('',#6129,#5358,#5359);
#4789=AXIS2_PLACEMENT_3D('',#6131,#5361,#5362);
#4790=AXIS2_PLACEMENT_3D('',#6135,#5365,#5366);
#4791=AXIS2_PLACEMENT_3D('',#6137,#5368,#5369);
#4792=AXIS2_PLACEMENT_3D('',#6139,#5370,#5371);
#4793=AXIS2_PLACEMENT_3D('',#6140,#5372,#5373);
#4794=AXIS2_PLACEMENT_3D('',#6141,#5374,#5375);
#4795=AXIS2_PLACEMENT_3D('',#6159,#5384,#5385);
#4796=AXIS2_PLACEMENT_3D('',#6161,#5386,#5387);
#4797=AXIS2_PLACEMENT_3D('',#6163,#5388,#5389);
#4798=AXIS2_PLACEMENT_3D('',#6165,#5390,#5391);
#4799=AXIS2_PLACEMENT_3D('',#6166,#5392,#5393);
#4800=AXIS2_PLACEMENT_3D('',#6167,#5394,#5395);
#4801=AXIS2_PLACEMENT_3D('',#6168,#5396,#5397);
#4802=AXIS2_PLACEMENT_3D('',#6169,#5398,#5399);
#4803=AXIS2_PLACEMENT_3D('',#6170,#5400,#5401);
#4804=AXIS2_PLACEMENT_3D('',#6171,#5402,#5403);
#4805=AXIS2_PLACEMENT_3D('',#6172,#5404,#5405);
#4806=AXIS2_PLACEMENT_3D('',#6173,#5406,#5407);
#4807=AXIS2_PLACEMENT_3D('',#6174,#5408,#5409);
#4808=AXIS2_PLACEMENT_3D('',#6175,#5410,#5411);
#4809=AXIS2_PLACEMENT_3D('',#6176,#5412,#5413);
#4810=AXIS2_PLACEMENT_3D('',#6177,#5414,#5415);
#4811=AXIS2_PLACEMENT_3D('',#6178,#5416,#5417);
#4812=AXIS2_PLACEMENT_3D('',#6179,#5418,#5419);
#4813=AXIS2_PLACEMENT_3D('',#6180,#5420,#5421);
#4814=AXIS2_PLACEMENT_3D('',#6181,#5422,#5423);
#4815=AXIS2_PLACEMENT_3D('',#6182,#5424,#5425);
#4816=AXIS2_PLACEMENT_3D('',#6183,#5426,#5427);
#4817=AXIS2_PLACEMENT_3D('',#6184,#5428,#5429);
#4818=AXIS2_PLACEMENT_3D('',#6185,#5430,#5431);
#4819=AXIS2_PLACEMENT_3D('',#6186,#5432,#5433);
#4820=AXIS2_PLACEMENT_3D('',#6187,#5434,#5435);
#4821=AXIS2_PLACEMENT_3D('',#6188,#5436,#5437);
#4822=AXIS2_PLACEMENT_3D('',#6189,#5438,#5439);
#4823=AXIS2_PLACEMENT_3D('',#6190,#5440,#5441);
#5208=DIRECTION('axis',(0.,0.,1.));
#5209=DIRECTION('refdir',(1.,0.,0.));
#5210=DIRECTION('center_axis',(0.,0.,-1.));
#5211=DIRECTION('ref_axis',(-1.,0.,0.));
#5212=DIRECTION('center_axis',(0.,0.,1.));
#5213=DIRECTION('ref_axis',(1.,0.,0.));
#5214=DIRECTION('center_axis',(0.,0.,1.));
#5215=DIRECTION('ref_axis',(1.,0.,0.));
#5216=DIRECTION('center_axis',(0.,0.,1.));
#5217=DIRECTION('ref_axis',(1.,0.,0.));
#5218=DIRECTION('center_axis',(0.,0.,1.));
#5219=DIRECTION('ref_axis',(1.,0.,0.));
#5220=DIRECTION('center_axis',(0.,0.,-1.));
#5221=DIRECTION('ref_axis',(1.,0.,0.));
#5222=DIRECTION('center_axis',(0.,0.,1.));
#5223=DIRECTION('ref_axis',(1.,0.,0.));
#5224=DIRECTION('center_axis',(0.,0.,-1.));
#5225=DIRECTION('ref_axis',(1.,0.,0.));
#5226=DIRECTION('center_axis',(0.,-1.,0.));
#5227=DIRECTION('ref_axis',(-1.,0.,0.));
#5228=DIRECTION('center_axis',(0.,0.,1.));
#5229=DIRECTION('ref_axis',(1.,0.,0.));
#5230=DIRECTION('center_axis',(0.,0.,1.));
#5231=DIRECTION('ref_axis',(1.,0.,0.));
#5232=DIRECTION('',(0.707106781186547,0.707106781186547,0.));
#5233=DIRECTION('',(1.,0.,0.));
#5234=DIRECTION('',(0.707106781186547,-0.707106781186547,0.));
#5235=DIRECTION('',(0.,-1.,0.));
#5236=DIRECTION('',(-0.707106781186547,-0.707106781186547,0.));
#5237=DIRECTION('',(-1.,0.,0.));
#5238=DIRECTION('',(-0.707106781186547,0.707106781186547,0.));
#5239=DIRECTION('',(0.,1.,0.));
#5240=DIRECTION('center_axis',(0.,0.,-1.));
#5241=DIRECTION('ref_axis',(1.,0.,0.));
#5242=DIRECTION('center_axis',(0.,0.,-1.));
#5243=DIRECTION('ref_axis',(1.,0.,0.));
#5244=DIRECTION('center_axis',(0.,0.,-1.));
#5245=DIRECTION('ref_axis',(1.,0.,0.));
#5246=DIRECTION('center_axis',(0.,0.,-1.));
#5247=DIRECTION('ref_axis',(1.,0.,0.));
#5248=DIRECTION('center_axis',(0.,0.,1.));
#5249=DIRECTION('ref_axis',(1.,0.,0.));
#5250=DIRECTION('',(0.,0.,1.));
#5251=DIRECTION('center_axis',(0.,0.,-1.));
#5252=DIRECTION('ref_axis',(1.,0.,0.));
#5253=DIRECTION('center_axis',(0.,0.,1.));
#5254=DIRECTION('ref_axis',(1.,0.,0.));
#5255=DIRECTION('center_axis',(0.,-1.,0.));
#5256=DIRECTION('ref_axis',(-1.,0.,0.));
#5257=DIRECTION('center_axis',(0.,0.,1.));
#5258=DIRECTION('ref_axis',(1.,0.,0.));
#5259=DIRECTION('center_axis',(0.,0.,1.));
#5260=DIRECTION('ref_axis',(1.,0.,0.));
#5261=DIRECTION('',(0.,0.,1.));
#5262=DIRECTION('center_axis',(0.,0.,-1.));
#5263=DIRECTION('ref_axis',(1.,0.,0.));
#5264=DIRECTION('center_axis',(0.,0.,-1.));
#5265=DIRECTION('ref_axis',(1.,0.,0.));
#5266=DIRECTION('center_axis',(0.,0.,1.));
#5267=DIRECTION('ref_axis',(1.,0.,0.));
#5268=DIRECTION('center_axis',(0.,-1.,0.));
#5269=DIRECTION('ref_axis',(-1.,0.,0.));
#5270=DIRECTION('center_axis',(0.,0.,1.));
#5271=DIRECTION('ref_axis',(1.,0.,0.));
#5272=DIRECTION('center_axis',(0.,0.,1.));
#5273=DIRECTION('ref_axis',(1.,0.,0.));
#5274=DIRECTION('',(0.,0.,1.));
#5275=DIRECTION('center_axis',(0.,0.,-1.));
#5276=DIRECTION('ref_axis',(1.,0.,0.));
#5277=DIRECTION('center_axis',(0.,0.,-1.));
#5278=DIRECTION('ref_axis',(1.,0.,0.));
#5279=DIRECTION('center_axis',(0.,0.,1.));
#5280=DIRECTION('ref_axis',(1.,0.,0.));
#5281=DIRECTION('center_axis',(1.22464679914735E-16,-1.,0.));
#5282=DIRECTION('ref_axis',(-1.,-1.22464679914735E-16,0.));
#5283=DIRECTION('center_axis',(0.,0.,1.));
#5284=DIRECTION('ref_axis',(1.,0.,0.));
#5285=DIRECTION('center_axis',(0.,-1.,0.));
#5286=DIRECTION('ref_axis',(-1.,0.,0.));
#5287=DIRECTION('center_axis',(0.,0.,1.));
#5288=DIRECTION('ref_axis',(1.,0.,0.));
#5289=DIRECTION('center_axis',(0.,0.,1.));
#5290=DIRECTION('ref_axis',(1.,0.,0.));
#5291=DIRECTION('',(0.,0.,1.));
#5292=DIRECTION('center_axis',(0.,0.,-1.));
#5293=DIRECTION('ref_axis',(1.,0.,0.));
#5294=DIRECTION('center_axis',(0.,0.,-1.));
#5295=DIRECTION('ref_axis',(1.,0.,0.));
#5296=DIRECTION('center_axis',(0.707106781186548,0.707106781186548,0.));
#5297=DIRECTION('ref_axis',(-0.499999999999996,0.499999999999996,-0.707106781186553));
#5298=DIRECTION('center_axis',(0.382683432365092,0.923879532511286,0.));
#5299=DIRECTION('ref_axis',(-0.923879532511286,0.382683432365092,0.));
#5300=DIRECTION('',(0.707106781186547,0.707106781186547,0.));
#5301=DIRECTION('center_axis',(0.923879532511283,0.382683432365099,3.39891166203448E-15));
#5302=DIRECTION('ref_axis',(-0.382683432365099,0.923879532511283,8.2056986317915E-15));
#5303=DIRECTION('center_axis',(0.,1.,0.));
#5304=DIRECTION('ref_axis',(-0.707106781186541,0.,-0.707106781186554));
#5305=DIRECTION('center_axis',(-0.382683432365099,0.923879532511283,3.39891166203448E-15));
#5306=DIRECTION('ref_axis',(-0.923879532511283,-0.382683432365099,8.2056986317915E-15));
#5307=DIRECTION('',(0.,1.,0.));
#5308=DIRECTION('center_axis',(-0.707106781186548,0.707106781186548,0.));
#5309=DIRECTION('ref_axis',(-0.499999999999996,-0.499999999999996,-0.707106781186553));
#5310=DIRECTION('center_axis',(-0.923879532511286,0.382683432365092,0.));
#5311=DIRECTION('ref_axis',(-0.382683432365092,-0.923879532511286,0.));
#5312=DIRECTION('',(-0.707106781186547,0.707106781186547,0.));
#5313=DIRECTION('center_axis',(-0.707106781186548,-0.707106781186548,0.));
#5314=DIRECTION('ref_axis',(0.499999999999996,-0.499999999999996,-0.707106781186553));
#5315=DIRECTION('center_axis',(-0.382683432365092,-0.923879532511286,0.));
#5316=DIRECTION('ref_axis',(0.923879532511286,-0.382683432365092,0.));
#5317=DIRECTION('',(-0.707106781186547,-0.707106781186547,0.));
#5318=DIRECTION('center_axis',(0.923879532511286,0.382683432365092,-8.20569863179153E-15));
#5319=DIRECTION('ref_axis',(-0.382683432365092,0.923879532511286,1.98103089256176E-14));
#5320=DIRECTION('center_axis',(0.,-1.,0.));
#5321=DIRECTION('ref_axis',(0.707106781186541,0.,-0.707106781186554));
#5322=DIRECTION('',(0.,-1.,0.));
#5323=DIRECTION('center_axis',(0.382683432365099,-0.923879532511283,3.39891166203448E-15));
#5324=DIRECTION('ref_axis',(0.923879532511283,0.382683432365099,8.2056986317915E-15));
#5325=DIRECTION('center_axis',(-1.,0.,0.));
#5326=DIRECTION('ref_axis',(0.,-0.707106781186541,-0.707106781186554));
#5327=DIRECTION('',(-1.,0.,0.));
#5328=DIRECTION('center_axis',(0.707106781186548,-0.707106781186548,0.));
#5329=DIRECTION('ref_axis',(0.499999999999996,0.499999999999996,-0.707106781186553));
#5330=DIRECTION('',(0.707106781186547,-0.707106781186547,0.));
#5331=DIRECTION('center_axis',(0.923879532511286,-0.382683432365092,0.));
#5332=DIRECTION('ref_axis',(0.382683432365092,0.923879532511286,0.));
#5333=DIRECTION('center_axis',(1.,0.,0.));
#5334=DIRECTION('ref_axis',(0.,0.707106781186541,-0.707106781186554));
#5335=DIRECTION('',(1.,0.,0.));
#5336=DIRECTION('center_axis',(-1.,0.,0.));
#5337=DIRECTION('ref_axis',(0.,-1.,0.));
#5338=DIRECTION('',(0.,0.,1.));
#5339=DIRECTION('',(0.,-1.,0.));
#5340=DIRECTION('',(0.,0.,1.));
#5341=DIRECTION('center_axis',(-0.707106781186548,-0.707106781186548,0.));
#5342=DIRECTION('ref_axis',(0.707106781186548,-0.707106781186548,0.));
#5343=DIRECTION('',(0.,0.,1.));
#5344=DIRECTION('',(0.707106781186547,-0.707106781186547,0.));
#5345=DIRECTION('center_axis',(0.,-1.,0.));
#5346=DIRECTION('ref_axis',(1.,0.,0.));
#5347=DIRECTION('',(0.,0.,1.));
#5348=DIRECTION('',(1.,0.,0.));
#5349=DIRECTION('center_axis',(0.707106781186548,-0.707106781186548,0.));
#5350=DIRECTION('ref_axis',(0.707106781186548,0.707106781186548,0.));
#5351=DIRECTION('',(0.,0.,1.));
#5352=DIRECTION('',(0.707106781186547,0.707106781186547,0.));
#5353=DIRECTION('center_axis',(0.707106781186548,0.707106781186548,0.));
#5354=DIRECTION('ref_axis',(-0.707106781186548,0.707106781186548,0.));
#5355=DIRECTION('',(0.,0.,1.));
#5356=DIRECTION('',(-0.707106781186547,0.707106781186547,0.));
#5357=DIRECTION('',(0.,0.,1.));
#5358=DIRECTION('center_axis',(1.,0.,0.));
#5359=DIRECTION('ref_axis',(0.,1.,0.));
#5360=DIRECTION('',(0.,1.,0.));
#5361=DIRECTION('center_axis',(0.,1.,0.));
#5362=DIRECTION('ref_axis',(-1.,0.,0.));
#5363=DIRECTION('',(0.,0.,1.));
#5364=DIRECTION('',(-1.,0.,0.));
#5365=DIRECTION('center_axis',(-0.707106781186548,0.707106781186548,0.));
#5366=DIRECTION('ref_axis',(-0.707106781186548,-0.707106781186548,0.));
#5367=DIRECTION('',(-0.707106781186547,-0.707106781186547,0.));
#5368=DIRECTION('center_axis',(0.,0.,-1.));
#5369=DIRECTION('ref_axis',(-1.,0.,0.));
#5370=DIRECTION('center_axis',(0.,0.,1.));
#5371=DIRECTION('ref_axis',(1.,0.,0.));
#5372=DIRECTION('center_axis',(0.,-1.,0.));
#5373=DIRECTION('ref_axis',(1.,0.,0.));
#5374=DIRECTION('center_axis',(0.,0.,1.));
#5375=DIRECTION('ref_axis',(1.,0.,0.));
#5376=DIRECTION('',(0.707106781186547,-0.707106781186547,0.));
#5377=DIRECTION('',(1.,0.,0.));
#5378=DIRECTION('',(0.707106781186547,0.707106781186547,0.));
#5379=DIRECTION('',(0.,1.,0.));
#5380=DIRECTION('',(-0.707106781186547,0.707106781186547,0.));
#5381=DIRECTION('',(-1.,0.,0.));
#5382=DIRECTION('',(-0.707106781186547,-0.707106781186547,0.));
#5383=DIRECTION('',(0.,-1.,0.));
#5384=DIRECTION('center_axis',(0.,0.,1.));
#5385=DIRECTION('ref_axis',(1.,0.,0.));
#5386=DIRECTION('center_axis',(0.,0.,1.));
#5387=DIRECTION('ref_axis',(1.,0.,0.));
#5388=DIRECTION('center_axis',(0.,0.,1.));
#5389=DIRECTION('ref_axis',(1.,0.,0.));
#5390=DIRECTION('center_axis',(0.,0.,1.));
#5391=DIRECTION('ref_axis',(1.,0.,0.));
#5392=DIRECTION('center_axis',(0.,0.,-1.));
#5393=DIRECTION('ref_axis',(-1.,0.,0.));
#5394=DIRECTION('center_axis',(0.,-1.,0.));
#5395=DIRECTION('ref_axis',(1.,0.,0.));
#5396=DIRECTION('center_axis',(0.,0.,-1.));
#5397=DIRECTION('ref_axis',(-1.,0.,0.));
#5398=DIRECTION('center_axis',(-1.22464679914735E-16,-1.,0.));
#5399=DIRECTION('ref_axis',(1.,-1.22464679914735E-16,0.));
#5400=DIRECTION('center_axis',(0.,0.,-1.));
#5401=DIRECTION('ref_axis',(-1.,0.,0.));
#5402=DIRECTION('center_axis',(0.,-1.,0.));
#5403=DIRECTION('ref_axis',(1.,0.,0.));
#5404=DIRECTION('center_axis',(0.707106781186548,-0.707106781186548,0.));
#5405=DIRECTION('ref_axis',(-0.5,-0.5,0.707106781186547));
#5406=DIRECTION('center_axis',(0.382683432365092,-0.923879532511286,8.20569863179167E-15));
#5407=DIRECTION('ref_axis',(-0.923879532511286,-0.382683432365092,1.98103089256179E-14));
#5408=DIRECTION('center_axis',(0.923879532511286,-0.382683432365092,0.));
#5409=DIRECTION('ref_axis',(-0.382683432365092,-0.923879532511286,0.));
#5410=DIRECTION('center_axis',(0.,-1.,0.));
#5411=DIRECTION('ref_axis',(-0.707106781186548,0.,0.707106781186548));
#5412=DIRECTION('center_axis',(-0.382683432365092,-0.923879532511286,0.));
#5413=DIRECTION('ref_axis',(-0.923879532511286,0.382683432365092,0.));
#5414=DIRECTION('center_axis',(-0.707106781186548,-0.707106781186548,0.));
#5415=DIRECTION('ref_axis',(-0.5,0.5,0.707106781186547));
#5416=DIRECTION('center_axis',(-0.923879532511286,-0.382683432365092,8.20569863179167E-15));
#5417=DIRECTION('ref_axis',(-0.382683432365092,0.923879532511286,1.98103089256179E-14));
#5418=DIRECTION('center_axis',(-0.707106781186548,0.707106781186548,0.));
#5419=DIRECTION('ref_axis',(0.5,0.5,0.707106781186547));
#5420=DIRECTION('center_axis',(-0.382683432365092,0.923879532511286,8.20569863179167E-15));
#5421=DIRECTION('ref_axis',(0.923879532511286,0.382683432365092,1.98103089256179E-14));
#5422=DIRECTION('center_axis',(0.923879532511286,-0.382683432365092,0.));
#5423=DIRECTION('ref_axis',(-0.382683432365092,-0.923879532511286,0.));
#5424=DIRECTION('center_axis',(0.,1.,0.));
#5425=DIRECTION('ref_axis',(0.707106781186548,0.,0.707106781186548));
#5426=DIRECTION('center_axis',(0.382683432365092,0.923879532511286,0.));
#5427=DIRECTION('ref_axis',(0.923879532511286,-0.382683432365092,0.));
#5428=DIRECTION('center_axis',(-1.,0.,0.));
#5429=DIRECTION('ref_axis',(0.,0.707106781186548,0.707106781186548));
#5430=DIRECTION('center_axis',(0.707106781186548,0.707106781186548,0.));
#5431=DIRECTION('ref_axis',(0.5,-0.5,0.707106781186547));
#5432=DIRECTION('center_axis',(0.923879532511286,0.382683432365092,8.20569863179167E-15));
#5433=DIRECTION('ref_axis',(0.382683432365092,-0.923879532511286,1.98103089256179E-14));
#5434=DIRECTION('center_axis',(1.,0.,0.));
#5435=DIRECTION('ref_axis',(0.,-0.707106781186548,0.707106781186548));
#5436=DIRECTION('center_axis',(0.,0.,1.));
#5437=DIRECTION('ref_axis',(1.,0.,0.));
#5438=DIRECTION('center_axis',(0.,-1.,0.));
#5439=DIRECTION('ref_axis',(-1.,0.,0.));
#5440=DIRECTION('center_axis',(0.,0.,1.));
#5441=DIRECTION('ref_axis',(1.,0.,0.));
#5442=DIRECTION('',(0.,0.,1.));
#5995=CARTESIAN_POINT('',(0.,0.,0.));
#5996=CARTESIAN_POINT('Origin',(20.5,0.,-54.5));
#5997=CARTESIAN_POINT('',(-20.5,-2.51052593825207E-15,-54.5));
#5998=CARTESIAN_POINT('Origin',(0.,0.,-54.5));
#5999=CARTESIAN_POINT('',(-20.,-2.44929359829471E-15,-54.5));
#6000=CARTESIAN_POINT('Origin',(0.,0.,-54.5));
#6001=CARTESIAN_POINT('Origin',(20.,0.,-37.5));
#6002=CARTESIAN_POINT('',(-20.5,-2.51052593825207E-15,-37.5));
#6003=CARTESIAN_POINT('Origin',(0.,0.,-37.5));
#6004=CARTESIAN_POINT('',(20.,-2.44929359829471E-15,-37.5));
#6005=CARTESIAN_POINT('Origin',(0.,0.,-37.5));
#6006=CARTESIAN_POINT('Origin',(23.5502525316942,-23.5502525316942,-54.5));
#6007=CARTESIAN_POINT('',(19.0502525316942,-23.5502525316942,-55.));
#6008=CARTESIAN_POINT('Origin',(23.5502525316942,-23.5502525316942,-55.));
#6009=CARTESIAN_POINT('',(19.5502525316942,-23.5502525316942,-54.5));
#6010=CARTESIAN_POINT('Origin',(19.0502525316942,-23.5502525316942,-54.5));
#6011=CARTESIAN_POINT('Origin',(23.5502525316942,-23.5502525316942,-54.5));
#6012=CARTESIAN_POINT('Origin',(0.,0.,-55.));
#6013=CARTESIAN_POINT('',(26.7928932188135,-29.5,-55.));
#6014=CARTESIAN_POINT('',(29.5,-26.7928932188135,-55.));
#6015=CARTESIAN_POINT('',(27.3964466094067,-28.8964466094067,-55.));
#6016=CARTESIAN_POINT('',(-26.7928932188135,-29.5,-55.));
#6017=CARTESIAN_POINT('',(-13.5,-29.5,-55.));
#6018=CARTESIAN_POINT('',(-29.5,-26.7928932188135,-55.));
#6019=CARTESIAN_POINT('',(-28.8964466094067,-27.3964466094067,-55.));
#6020=CARTESIAN_POINT('',(-29.5,26.7928932188135,-55.));
#6021=CARTESIAN_POINT('',(-29.5,13.5,-55.));
#6022=CARTESIAN_POINT('',(-26.7928932188135,29.5,-55.));
#6023=CARTESIAN_POINT('',(-27.3964466094067,28.8964466094067,-55.));
#6024=CARTESIAN_POINT('',(26.7928932188135,29.5,-55.));
#6025=CARTESIAN_POINT('',(13.5,29.5,-55.));
#6026=CARTESIAN_POINT('',(29.5,26.7928932188135,-55.));
#6027=CARTESIAN_POINT('',(28.8964466094067,27.3964466094067,-55.));
#6028=CARTESIAN_POINT('',(29.5,-13.5,-55.));
#6029=CARTESIAN_POINT('',(-28.0502525316942,23.5502525316942,-55.));
#6030=CARTESIAN_POINT('Origin',(-23.5502525316942,23.5502525316942,-55.));
#6031=CARTESIAN_POINT('',(-20.5,2.51052593825207E-15,-55.));
#6032=CARTESIAN_POINT('Origin',(0.,0.,-55.));
#6033=CARTESIAN_POINT('',(19.0502525316942,23.5502525316942,-55.));
#6034=CARTESIAN_POINT('Origin',(23.5502525316942,23.5502525316942,-55.));
#6035=CARTESIAN_POINT('',(-28.0502525316942,-23.5502525316942,-55.));
#6036=CARTESIAN_POINT('Origin',(-23.5502525316942,-23.5502525316942,-55.));
#6037=CARTESIAN_POINT('Origin',(23.5502525316942,-23.5502525316942,-50.));
#6038=CARTESIAN_POINT('',(19.5502525316942,-23.5502525316942,-37.5));
#6039=CARTESIAN_POINT('',(19.5502525316942,-23.5502525316942,-50.));
#6040=CARTESIAN_POINT('Origin',(23.5502525316942,-23.5502525316942,-37.5));
#6041=CARTESIAN_POINT('Origin',(-23.5502525316942,23.5502525316942,-54.5));
#6042=CARTESIAN_POINT('',(-27.5502525316942,23.5502525316942,-54.5));
#6043=CARTESIAN_POINT('Origin',(-28.0502525316942,23.5502525316942,-54.5));
#6044=CARTESIAN_POINT('Origin',(-23.5502525316942,23.5502525316942,-54.5));
#6045=CARTESIAN_POINT('Origin',(-23.5502525316942,23.5502525316942,-50.));
#6046=CARTESIAN_POINT('',(-27.5502525316942,23.5502525316942,-37.5));
#6047=CARTESIAN_POINT('',(-27.5502525316942,23.5502525316942,-50.));
#6048=CARTESIAN_POINT('',(-19.5502525316942,23.5502525316942,-37.5));
#6049=CARTESIAN_POINT('Origin',(-23.5502525316942,23.5502525316942,-37.5));
#6050=CARTESIAN_POINT('Origin',(-23.5502525316942,23.5502525316942,-37.5));
#6051=CARTESIAN_POINT('Origin',(-23.5502525316942,-23.5502525316942,-54.5));
#6052=CARTESIAN_POINT('',(-27.5502525316942,-23.5502525316942,-54.5));
#6053=CARTESIAN_POINT('Origin',(-28.0502525316942,-23.5502525316942,-54.5));
#6054=CARTESIAN_POINT('Origin',(-23.5502525316942,-23.5502525316942,-54.5));
#6055=CARTESIAN_POINT('Origin',(-23.5502525316942,-23.5502525316942,-50.));
#6056=CARTESIAN_POINT('',(-27.5502525316942,-23.5502525316942,-37.5));
#6057=CARTESIAN_POINT('',(-27.5502525316942,-23.5502525316942,-50.));
#6058=CARTESIAN_POINT('',(-19.5502525316942,-23.5502525316942,-37.5));
#6059=CARTESIAN_POINT('Origin',(-23.5502525316942,-23.5502525316942,-37.5));
#6060=CARTESIAN_POINT('Origin',(-23.5502525316942,-23.5502525316942,-37.5));
#6061=CARTESIAN_POINT('Origin',(0.,0.,-54.5));
#6062=CARTESIAN_POINT('Origin',(-20.5,-2.51052593825207E-15,-54.5));
#6063=CARTESIAN_POINT('Origin',(23.5502525316942,23.5502525316942,-54.5));
#6064=CARTESIAN_POINT('',(19.5502525316942,23.5502525316942,-54.5));
#6065=CARTESIAN_POINT('Origin',(19.0502525316942,23.5502525316942,-54.5));
#6066=CARTESIAN_POINT('Origin',(23.5502525316942,23.5502525316942,-54.5));
#6067=CARTESIAN_POINT('Origin',(23.5502525316942,23.5502525316942,-50.));
#6068=CARTESIAN_POINT('',(19.5502525316942,23.5502525316942,-37.5));
#6069=CARTESIAN_POINT('',(19.5502525316942,23.5502525316942,-50.));
#6070=CARTESIAN_POINT('',(27.5502525316942,23.5502525316942,-37.5));
#6071=CARTESIAN_POINT('Origin',(23.5502525316942,23.5502525316942,-37.5));
#6072=CARTESIAN_POINT('Origin',(23.5502525316942,23.5502525316942,-37.5));
#6073=CARTESIAN_POINT('Origin',(-27.3964466094067,28.8964466094067,-54.5));
#6074=CARTESIAN_POINT('',(-30.,27.,-54.5));
#6075=CARTESIAN_POINT('Origin',(-29.5,26.7928932188135,-54.5));
#6076=CARTESIAN_POINT('',(-27.,30.,-54.5));
#6077=CARTESIAN_POINT('',(-27.75,29.25,-54.5));
#6078=CARTESIAN_POINT('Origin',(-26.7928932188135,29.5,-54.5));
#6079=CARTESIAN_POINT('Origin',(-29.5,13.5,-54.5));
#6080=CARTESIAN_POINT('',(-30.,-27.,-54.5));
#6081=CARTESIAN_POINT('Origin',(-29.5,-26.7928932188135,-54.5));
#6082=CARTESIAN_POINT('',(-30.,13.5,-54.5));
#6083=CARTESIAN_POINT('Origin',(-28.8964466094067,-27.3964466094067,-54.5));
#6084=CARTESIAN_POINT('',(-27.,-30.,-54.5));
#6085=CARTESIAN_POINT('Origin',(-26.7928932188135,-29.5,-54.5));
#6086=CARTESIAN_POINT('',(-29.25,-27.75,-54.5));
#6087=CARTESIAN_POINT('Origin',(27.3964466094067,-28.8964466094067,-54.5));
#6088=CARTESIAN_POINT('',(30.,-27.,-54.5));
#6089=CARTESIAN_POINT('Origin',(29.5,-26.7928932188135,-54.5));
#6090=CARTESIAN_POINT('',(27.,-30.,-54.5));
#6091=CARTESIAN_POINT('',(27.75,-29.25,-54.5));
#6092=CARTESIAN_POINT('Origin',(26.7928932188135,-29.5,-54.5));
#6093=CARTESIAN_POINT('Origin',(29.5,-13.5,-54.5));
#6094=CARTESIAN_POINT('',(30.,27.,-54.5));
#6095=CARTESIAN_POINT('',(30.,-13.5,-54.5));
#6096=CARTESIAN_POINT('Origin',(29.5,26.7928932188135,-54.5));
#6097=CARTESIAN_POINT('Origin',(-13.5,-29.5,-54.5));
#6098=CARTESIAN_POINT('',(-13.5,-30.,-54.5));
#6099=CARTESIAN_POINT('Origin',(28.8964466094067,27.3964466094067,-54.5));
#6100=CARTESIAN_POINT('',(27.,30.,-54.5));
#6101=CARTESIAN_POINT('',(29.25,27.75,-54.5));
#6102=CARTESIAN_POINT('Origin',(26.7928932188135,29.5,-54.5));
#6103=CARTESIAN_POINT('Origin',(13.5,29.5,-54.5));
#6104=CARTESIAN_POINT('',(13.5,30.,-54.5));
#6105=CARTESIAN_POINT('Origin',(-30.,27.,-50.));
#6106=CARTESIAN_POINT('',(-30.,-27.,-37.5));
#6107=CARTESIAN_POINT('',(-30.,-27.,-50.));
#6108=CARTESIAN_POINT('',(-30.,27.,-37.5));
#6109=CARTESIAN_POINT('',(-30.,13.5,-37.5));
#6110=CARTESIAN_POINT('',(-30.,27.,-50.));
#6111=CARTESIAN_POINT('Origin',(-30.,-27.,-50.));
#6112=CARTESIAN_POINT('',(-27.,-30.,-37.5));
#6113=CARTESIAN_POINT('',(-27.,-30.,-50.));
#6114=CARTESIAN_POINT('',(-29.25,-27.75,-37.5));
#6115=CARTESIAN_POINT('Origin',(-27.,-30.,-50.));
#6116=CARTESIAN_POINT('',(27.,-30.,-37.5));
#6117=CARTESIAN_POINT('',(27.,-30.,-50.));
#6118=CARTESIAN_POINT('',(-13.5,-30.,-37.5));
#6119=CARTESIAN_POINT('Origin',(27.,-30.,-50.));
#6120=CARTESIAN_POINT('',(30.,-27.,-37.5));
#6121=CARTESIAN_POINT('',(30.,-27.,-50.));
#6122=CARTESIAN_POINT('',(27.75,-29.25,-37.5));
#6123=CARTESIAN_POINT('Origin',(30.,27.,-50.));
#6124=CARTESIAN_POINT('',(27.,30.,-37.5));
#6125=CARTESIAN_POINT('',(27.,30.,-50.));
#6126=CARTESIAN_POINT('',(30.,27.,-37.5));
#6127=CARTESIAN_POINT('',(29.25,27.75,-37.5));
#6128=CARTESIAN_POINT('',(30.,27.,-50.));
#6129=CARTESIAN_POINT('Origin',(30.,-27.,-50.));
#6130=CARTESIAN_POINT('',(30.,-13.5,-37.5));
#6131=CARTESIAN_POINT('Origin',(27.,30.,-50.));
#6132=CARTESIAN_POINT('',(-27.,30.,-37.5));
#6133=CARTESIAN_POINT('',(-27.,30.,-50.));
#6134=CARTESIAN_POINT('',(13.5,30.,-37.5));
#6135=CARTESIAN_POINT('Origin',(-27.,30.,-50.));
#6136=CARTESIAN_POINT('',(-27.75,29.25,-37.5));
#6137=CARTESIAN_POINT('Origin',(-23.5502525316942,23.5502525316942,-37.5));
#6138=CARTESIAN_POINT('',(-19.0502525316942,23.5502525316942,-37.));
#6139=CARTESIAN_POINT('Origin',(-23.5502525316942,23.5502525316942,-37.));
#6140=CARTESIAN_POINT('Origin',(-19.0502525316942,23.5502525316942,-37.5));
#6141=CARTESIAN_POINT('Origin',(0.,0.,-37.));
#6142=CARTESIAN_POINT('',(26.7928932188135,29.5,-37.));
#6143=CARTESIAN_POINT('',(29.5,26.7928932188135,-37.));
#6144=CARTESIAN_POINT('',(28.8964466094067,27.3964466094067,-37.));
#6145=CARTESIAN_POINT('',(-26.7928932188135,29.5,-37.));
#6146=CARTESIAN_POINT('',(13.5,29.5,-37.));
#6147=CARTESIAN_POINT('',(-29.5,26.7928932188135,-37.));
#6148=CARTESIAN_POINT('',(-27.3964466094067,28.8964466094067,-37.));
#6149=CARTESIAN_POINT('',(-29.5,-26.7928932188135,-37.));
#6150=CARTESIAN_POINT('',(-29.5,13.5,-37.));
#6151=CARTESIAN_POINT('',(-26.7928932188135,-29.5,-37.));
#6152=CARTESIAN_POINT('',(-28.8964466094067,-27.3964466094067,-37.));
#6153=CARTESIAN_POINT('',(26.7928932188135,-29.5,-37.));
#6154=CARTESIAN_POINT('',(-13.5,-29.5,-37.));
#6155=CARTESIAN_POINT('',(29.5,-26.7928932188135,-37.));
#6156=CARTESIAN_POINT('',(27.3964466094067,-28.8964466094067,-37.));
#6157=CARTESIAN_POINT('',(29.5,-13.5,-37.));
#6158=CARTESIAN_POINT('',(-19.0502525316942,-23.5502525316942,-37.));
#6159=CARTESIAN_POINT('Origin',(-23.5502525316942,-23.5502525316942,-37.));
#6160=CARTESIAN_POINT('',(28.0502525316942,23.5502525316942,-37.));
#6161=CARTESIAN_POINT('Origin',(23.5502525316942,23.5502525316942,-37.));
#6162=CARTESIAN_POINT('',(19.0502525316942,-23.5502525316942,-37.));
#6163=CARTESIAN_POINT('Origin',(23.5502525316942,-23.5502525316942,-37.));
#6164=CARTESIAN_POINT('',(20.5,-2.51052593825207E-15,-37.));
#6165=CARTESIAN_POINT('Origin',(0.,0.,-37.));
#6166=CARTESIAN_POINT('Origin',(-23.5502525316942,-23.5502525316942,-37.5));
#6167=CARTESIAN_POINT('Origin',(-19.0502525316942,-23.5502525316942,-37.5));
#6168=CARTESIAN_POINT('Origin',(0.,0.,-37.5));
#6169=CARTESIAN_POINT('Origin',(20.5,-2.51052593825207E-15,-37.5));
#6170=CARTESIAN_POINT('Origin',(23.5502525316942,23.5502525316942,-37.5));
#6171=CARTESIAN_POINT('Origin',(28.0502525316942,23.5502525316942,-37.5));
#6172=CARTESIAN_POINT('Origin',(-28.8964466094067,-27.3964466094067,-37.5));
#6173=CARTESIAN_POINT('Origin',(-29.5,-26.7928932188135,-37.5));
#6174=CARTESIAN_POINT('Origin',(-26.7928932188135,-29.5,-37.5));
#6175=CARTESIAN_POINT('Origin',(-29.5,13.5,-37.5));
#6176=CARTESIAN_POINT('Origin',(-29.5,26.7928932188135,-37.5));
#6177=CARTESIAN_POINT('Origin',(-27.3964466094067,28.8964466094067,-37.5));
#6178=CARTESIAN_POINT('Origin',(-26.7928932188135,29.5,-37.5));
#6179=CARTESIAN_POINT('Origin',(28.8964466094067,27.3964466094067,-37.5));
#6180=CARTESIAN_POINT('Origin',(29.5,26.7928932188135,-37.5));
#6181=CARTESIAN_POINT('Origin',(26.7928932188135,29.5,-37.5));
#6182=CARTESIAN_POINT('Origin',(29.5,-13.5,-37.5));
#6183=CARTESIAN_POINT('Origin',(29.5,-26.7928932188135,-37.5));
#6184=CARTESIAN_POINT('Origin',(13.5,29.5,-37.5));
#6185=CARTESIAN_POINT('Origin',(27.3964466094067,-28.8964466094067,-37.5));
#6186=CARTESIAN_POINT('Origin',(26.7928932188135,-29.5,-37.5));
#6187=CARTESIAN_POINT('Origin',(-13.5,-29.5,-37.5));
#6188=CARTESIAN_POINT('Origin',(23.5502525316942,-23.5502525316942,-37.5));
#6189=CARTESIAN_POINT('Origin',(19.0502525316942,-23.5502525316942,-37.5));
#6190=CARTESIAN_POINT('Origin',(0.,0.,-46.));
#6191=CARTESIAN_POINT('',(-20.5,-2.51052593825207E-15,-46.));
#74094=UNCERTAINTY_MEASURE_WITH_UNIT(LENGTH_MEASURE(0.01),#74104,
'DISTANCE_ACCURACY_VALUE',
'Maximum model space distance between geometric entities at asserted c
onnectivities');
#74097=UNCERTAINTY_MEASURE_WITH_UNIT(LENGTH_MEASURE(0.01),#74104,
'DISTANCE_ACCURACY_VALUE',
'Maximum model space distance between geometric entities at asserted c
onnectivities');
#74100=(
GEOMETRIC_REPRESENTATION_CONTEXT(3)
GLOBAL_UNCERTAINTY_ASSIGNED_CONTEXT((#74094))
GLOBAL_UNIT_ASSIGNED_CONTEXT((#74104,#74106,#74107))
REPRESENTATION_CONTEXT('','3D')
);
#74103=(
GEOMETRIC_REPRESENTATION_CONTEXT(3)
GLOBAL_UNCERTAINTY_ASSIGNED_CONTEXT((#74097))
GLOBAL_UNIT_ASSIGNED_CONTEXT((#74104,#74106,#74107))
REPRESENTATION_CONTEXT('','3D')
);
#74104=(
LENGTH_UNIT()
NAMED_UNIT(*)
SI_UNIT(.MILLI.,.METRE.)
);
#74106=(
NAMED_UNIT(*)
PLANE_ANGLE_UNIT()
SI_UNIT($,.RADIAN.)
);
#74107=(
NAMED_UNIT(*)
SI_UNIT($,.STERADIAN.)
SOLID_ANGLE_UNIT()
);
#74110=SHAPE_DEFINITION_REPRESENTATION(#74115,#74129);
#74115=PRODUCT_DEFINITION_SHAPE('',$,#74135);
#74129=SHAPE_REPRESENTATION('',(#4729),#74100);
#74132=PRODUCT_DEFINITION_CONTEXT('part definition',#74149,'design');
#74135=PRODUCT_DEFINITION('base','Base',#74140,#74132);
#74140=PRODUCT_DEFINITION_FORMATION('',$,#74153);
#74149=APPLICATION_CONTEXT(
'Core Data for Automotive Mechanical Design Process');
#74150=PRODUCT_CONTEXT('part definition',#74149,'mechanical');
#74153=PRODUCT('base','Base',$,(#74150));
#74157=PRESENTATION_STYLE_ASSIGNMENT((#74161));
#74161=SURFACE_STYLE_USAGE(.BOTH.,#74165);
#74165=SURFACE_SIDE_STYLE('',(#74169));
#74169=SURFACE_STYLE_FILL_AREA(#74173);
#74173=FILL_AREA_STYLE('Opaque(55,55,55)',(#74177));
#74177=FILL_AREA_STYLE_COLOUR('Opaque(55,55,55)',#74181);
#74181=COLOUR_RGB('Opaque(55,55,55)', 0.09019608, 0.27058824, 0.51372549);
ENDSEC;
END-ISO-10303-21;
